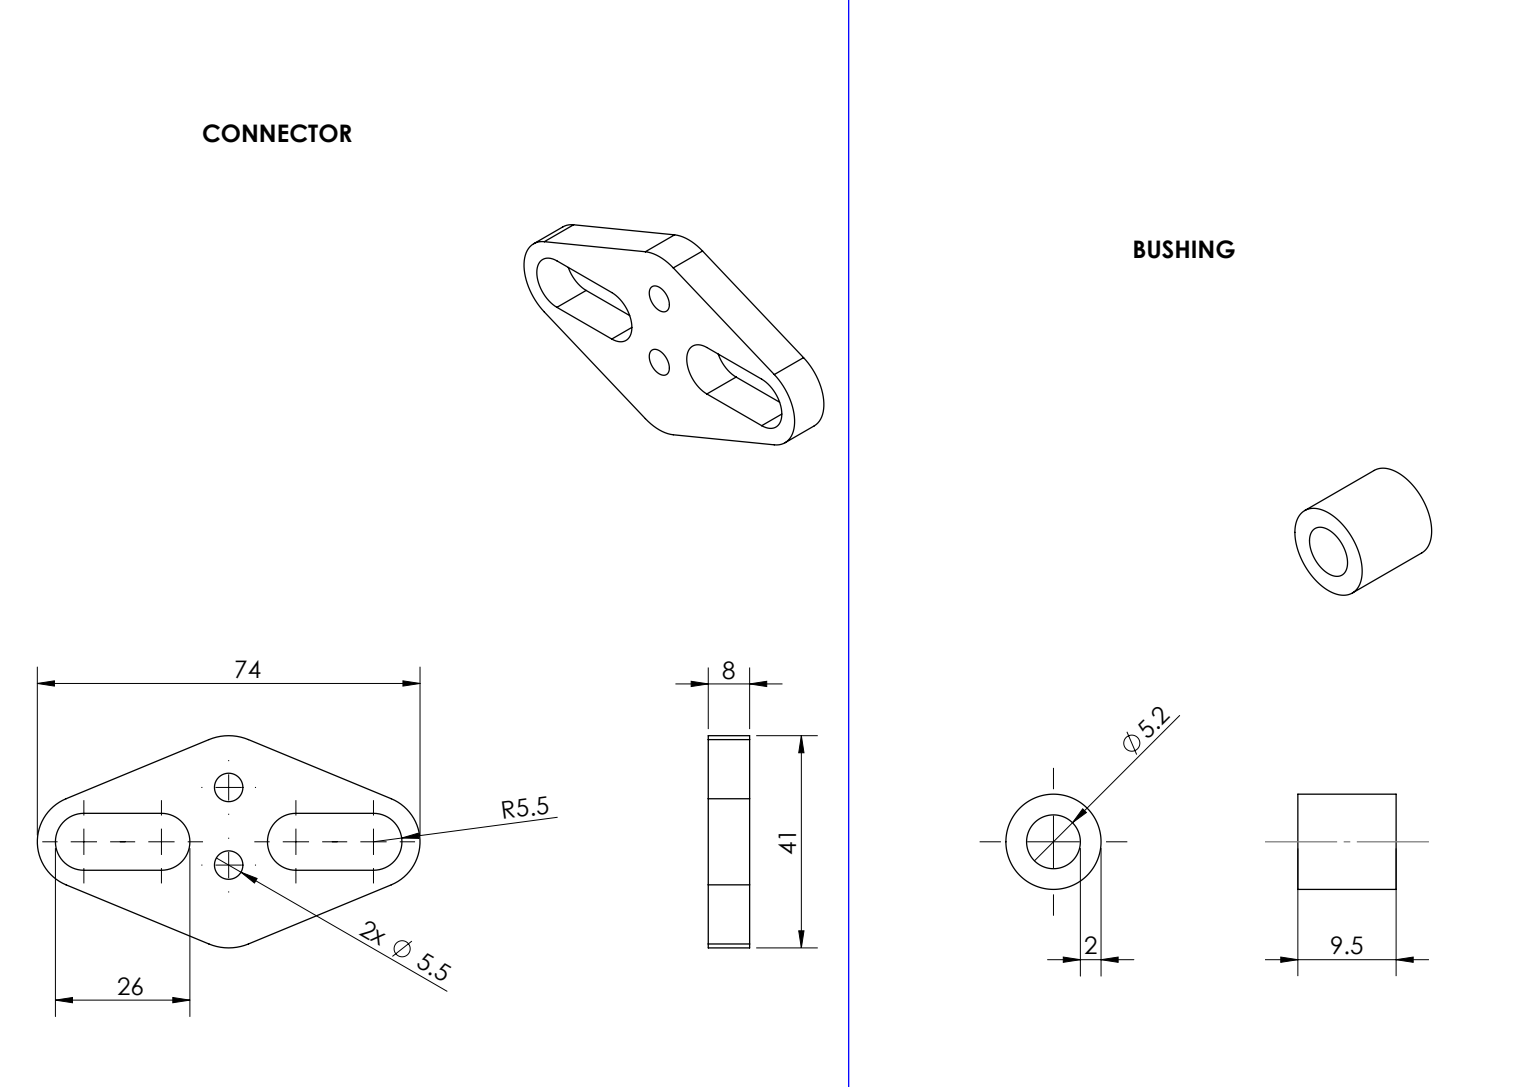
ISO-10303-21;
HEADER;
FILE_DESCRIPTION (('STEP AP214'),
    '1' );
FILE_NAME ('bushing.step',
    '2026-09-24T10:26:00',
    ( '' ),
    ( '' ),
    'SwSTEP 2.0',
    'SolidWorks 2026',
    '' );
FILE_SCHEMA (( 'AUTOMOTIVE_DESIGN' ));
ENDSEC;

DATA;
#17=EDGE_CURVE ( 'NONE', #13288, #10667, #2123, .T. ) ;
#63=PRODUCT ( 'bushing', 'bushing', '', ( #1978 ) ) ;
#90=SURFACE_STYLE_FILL_AREA ( #4690 ) ;
#131=VERTEX_POINT ( 'NONE', #10090 ) ;
#167=CARTESIAN_POINT ( 'NONE',  ( 0.000000000000000000, 0.000000000000000000, 0.000000000000000000 ) ) ;
#198=LINE ( 'NONE', #5806, #5338 ) ;
#221=AXIS2_PLACEMENT_3D ( 'NONE', #6634, #1226, #3433 ) ;
#307=UNCERTAINTY_MEASURE_WITH_UNIT (LENGTH_MEASURE( 1.000000000000000082E-05 ), #6803, 'distance_accuracy_value', 'NONE');
#327=EDGE_CURVE ( 'NONE', #12296, #10667, #14351, .T. ) ;
#475=SURFACE_STYLE_FILL_AREA ( #10569 ) ;
#957=AXIS2_PLACEMENT_3D ( 'NONE', #1843, #13854, #8266 ) ;
#1044=PRODUCT_DEFINITION_CONTEXT ( 'detailed design', #12786, 'design' ) ;
#1088=EDGE_CURVE ( 'NONE', #10667, #12296, #12886, .T. ) ;
#1201=( GEOMETRIC_REPRESENTATION_CONTEXT ( 3 ) GLOBAL_UNCERTAINTY_ASSIGNED_CONTEXT ( ( #8054 ) ) GLOBAL_UNIT_ASSIGNED_CONTEXT ( ( #10718, #4082, #12760 ) ) REPRESENTATION_CONTEXT ( 'NONE', 'WORKASPACE' ) );
#1226=DIRECTION ( 'NONE',  ( 0.000000000000000000, 0.000000000000000000, -1.000000000000000000 ) ) ;
#1235=EDGE_CURVE ( 'NONE', #14042, #13288, #9119, .T. ) ;
#1400=SHAPE_REPRESENTATION ( 'bushing', ( #11025 ), #4496 ) ;
#1424=AXIS2_PLACEMENT_3D ( 'NONE', #12440, #8035, #12508 ) ;
#1490=PLANE ( 'NONE',  #4984 ) ;
#1555=EDGE_CURVE ( 'NONE', #8738, #12036, #8933, .T. ) ;
#1727=EDGE_CURVE ( 'NONE', #8738, #13954, #7266, .T. ) ;
#1833=CYLINDRICAL_SURFACE ( 'NONE', #4021, 4.599999999999999645 ) ;
#1843=CARTESIAN_POINT ( 'NONE',  ( 28.00000000000000355, 29.99999999999999645, -34.50000000000000000 ) ) ;
#1978=PRODUCT_CONTEXT ( 'NONE', #7358, 'mechanical' ) ;
#1980=DIRECTION ( 'NONE',  ( 0.000000000000000000, 0.000000000000000000, -1.000000000000000000 ) ) ;
#2067=DIRECTION ( 'NONE',  ( -1.000000000000000000, 0.000000000000000000, 0.000000000000000000 ) ) ;
#2122=ORIENTED_EDGE ( 'NONE', *, *, #327, .F. ) ;
#2123=LINE ( 'NONE', #12076, #5253 ) ;
#2130=CARTESIAN_POINT ( 'NONE',  ( 30.60000000000000853, 29.99999999999999645, -24.99999999999999289 ) ) ;
#2532=ORIENTED_EDGE ( 'NONE', *, *, #4053, .F. ) ;
#2637=FACE_OUTER_BOUND ( 'NONE', #10692, .T. ) ;
#2660=CARTESIAN_POINT ( 'NONE',  ( 32.60000000000000142, 29.99999999999999645, -34.50000000000000000 ) ) ;
#2840=DIRECTION ( 'NONE',  ( 0.000000000000000000, 0.000000000000000000, -1.000000000000000000 ) ) ;
#2852=STYLED_ITEM ( 'NONE', ( #9618 ), #11938 ) ;
#2947=CARTESIAN_POINT ( 'NONE',  ( 28.00000000000000355, 29.99999999999999645, -34.50000000000000000 ) ) ;
#3172=EDGE_CURVE ( 'NONE', #14042, #12296, #5144, .T. ) ;
#3238=CARTESIAN_POINT ( 'NONE',  ( 23.40000000000000213, 29.99999999999999645, -24.99999999999999289 ) ) ;
#3381=( GEOMETRIC_REPRESENTATION_CONTEXT ( 3 ) GLOBAL_UNCERTAINTY_ASSIGNED_CONTEXT ( ( #307 ) ) GLOBAL_UNIT_ASSIGNED_CONTEXT ( ( #6803, #13337, #12303 ) ) REPRESENTATION_CONTEXT ( 'NONE', 'WORKASPACE' ) );
#3390=SURFACE_SIDE_STYLE ('',( #90 ) ) ;
#3399=DIRECTION ( 'NONE',  ( 0.000000000000000000, 0.000000000000000000, 1.000000000000000000 ) ) ;
#3433=DIRECTION ( 'NONE',  ( -1.000000000000000000, 0.000000000000000000, 0.000000000000000000 ) ) ;
#3454=FILL_AREA_STYLE_COLOUR ( '', #12640 ) ;
#3476=ADVANCED_FACE ( 'NONE', ( #3864, #3644 ), #3788, .F. ) ;
#3545=ORIENTED_EDGE ( 'NONE', *, *, #1555, .T. ) ;
#3554=UNCERTAINTY_MEASURE_WITH_UNIT (LENGTH_MEASURE( 1.000000000000000082E-05 ), #6295, 'distance_accuracy_value', 'NONE');
#3644=FACE_BOUND ( 'NONE', #8759, .T. ) ;
#3688=CARTESIAN_POINT ( 'NONE',  ( 28.00000000000000355, 29.99999999999999645, -24.99999999999999289 ) ) ;
#3750=ADVANCED_FACE ( 'NONE', ( #7708, #3845 ), #1490, .T. ) ;
#3788=PLANE ( 'NONE',  #5864 ) ;
#3845=FACE_BOUND ( 'NONE', #6428, .T. ) ;
#3864=FACE_OUTER_BOUND ( 'NONE', #10022, .T. ) ;
#3952=ORIENTED_EDGE ( 'NONE', *, *, #17, .T. ) ;
#3999=EDGE_LOOP ( 'NONE', ( #5182, #7262, #9638, #5982 ) ) ;
#4021=AXIS2_PLACEMENT_3D ( 'NONE', #2947, #8699, #12005 ) ;
#4053=EDGE_CURVE ( 'NONE', #12036, #131, #12295, .T. ) ;
#4076=DIRECTION ( 'NONE',  ( 1.000000000000000000, 0.000000000000000000, 0.000000000000000000 ) ) ;
#4082=( NAMED_UNIT ( * ) PLANE_ANGLE_UNIT ( ) SI_UNIT ( $, .RADIAN. ) );
#4139=CARTESIAN_POINT ( 'NONE',  ( 28.00000000000000355, 29.99999999999999645, -34.50000000000000000 ) ) ;
#4242=DIRECTION ( 'NONE',  ( 0.000000000000000000, 0.000000000000000000, -1.000000000000000000 ) ) ;
#4416=ORIENTED_EDGE ( 'NONE', *, *, #4053, .T. ) ;
#4496=( GEOMETRIC_REPRESENTATION_CONTEXT ( 3 ) GLOBAL_UNCERTAINTY_ASSIGNED_CONTEXT ( ( #3554 ) ) GLOBAL_UNIT_ASSIGNED_CONTEXT ( ( #6295, #13197, #5205 ) ) REPRESENTATION_CONTEXT ( 'NONE', 'WORKASPACE' ) );
#4503=DIRECTION ( 'NONE',  ( -1.000000000000000000, 0.000000000000000000, 0.000000000000000000 ) ) ;
#4611=VECTOR ( 'NONE', #10707, 1000.000000000000000 ) ;
#4642=AXIS2_PLACEMENT_3D ( 'NONE', #7297, #4242, #11772 ) ;
#4670=DIRECTION ( 'NONE',  ( 0.000000000000000000, 0.000000000000000000, 1.000000000000000000 ) ) ;
#4690=FILL_AREA_STYLE ('',( #3454 ) ) ;
#4870=ORIENTED_EDGE ( 'NONE', *, *, #1088, .F. ) ;
#4945=ORIENTED_EDGE ( 'NONE', *, *, #3172, .F. ) ;
#4984=AXIS2_PLACEMENT_3D ( 'NONE', #5856, #5933, #12751 ) ;
#5009=CARTESIAN_POINT ( 'NONE',  ( 28.00000000000000355, 29.99999999999999645, -34.50000000000000000 ) ) ;
#5142=DIRECTION ( 'NONE',  ( 0.000000000000000000, 0.000000000000000000, -1.000000000000000000 ) ) ;
#5144=LINE ( 'NONE', #11885, #4611 ) ;
#5155=AXIS2_PLACEMENT_3D ( 'NONE', #5009, #14095, #4076 ) ;
#5181=DIRECTION ( 'NONE',  ( -1.000000000000000000, 0.000000000000000000, 0.000000000000000000 ) ) ;
#5182=ORIENTED_EDGE ( 'NONE', *, *, #1555, .F. ) ;
#5205=( NAMED_UNIT ( * ) SI_UNIT ( $, .STERADIAN. ) SOLID_ANGLE_UNIT ( ) );
#5252=DIRECTION ( 'NONE',  ( 0.000000000000000000, 0.000000000000000000, 1.000000000000000000 ) ) ;
#5253=VECTOR ( 'NONE', #13119, 1000.000000000000000 ) ;
#5338=VECTOR ( 'NONE', #4670, 1000.000000000000000 ) ;
#5441=DIRECTION ( 'NONE',  ( 1.000000000000000000, 0.000000000000000000, 0.000000000000000000 ) ) ;
#5457=AXIS2_PLACEMENT_3D ( 'NONE', #6271, #7371, #5181 ) ;
#5565=ADVANCED_BREP_SHAPE_REPRESENTATION ( '', ( #11938, #11025 ), #4496 ) ;
#5623=AXIS2_PLACEMENT_3D ( 'NONE', #4139, #5142, #2067 ) ;
#5752=CYLINDRICAL_SURFACE ( 'NONE', #1424, 2.600000000000004974 ) ;
#5806=CARTESIAN_POINT ( 'NONE',  ( 32.60000000000000142, 29.99999999999999645, -34.50000000000000000 ) ) ;
#5856=CARTESIAN_POINT ( 'NONE',  ( 28.00000000000000355, 29.99999999999999645, -34.50000000000000000 ) ) ;
#5864=AXIS2_PLACEMENT_3D ( 'NONE', #8298, #2840, #12549 ) ;
#5915=MECHANICAL_DESIGN_GEOMETRIC_PRESENTATION_REPRESENTATION('',(#12250),#3381);
#5933=DIRECTION ( 'NONE',  ( 0.000000000000000000, 0.000000000000000000, -1.000000000000000000 ) ) ;
#5982=ORIENTED_EDGE ( 'NONE', *, *, #6678, .T. ) ;
#6199=ADVANCED_FACE ( 'NONE', ( #8434 ), #8281, .F. ) ;
#6271=CARTESIAN_POINT ( 'NONE',  ( 28.00000000000000355, 29.99999999999999645, -24.99999999999999289 ) ) ;
#6295=( LENGTH_UNIT ( ) NAMED_UNIT ( * ) SI_UNIT ( .MILLI., .METRE. ) );
#6337=ORIENTED_EDGE ( 'NONE', *, *, #6678, .F. ) ;
#6353=SHAPE_DEFINITION_REPRESENTATION ( #13869, #1400 ) ;
#6355=CARTESIAN_POINT ( 'NONE',  ( 28.00000000000000355, 29.99999999999999645, -34.50000000000000000 ) ) ;
#6428=EDGE_LOOP ( 'NONE', ( #11229, #10714 ) ) ;
#6470=CARTESIAN_POINT ( 'NONE',  ( 28.00000000000000355, 29.99999999999999645, -34.50000000000000000 ) ) ;
#6497=CIRCLE ( 'NONE', #4642, 2.600000000000004974 ) ;
#6524=DIRECTION ( 'NONE',  ( 0.000000000000000000, 0.000000000000000000, 1.000000000000000000 ) ) ;
#6634=CARTESIAN_POINT ( 'NONE',  ( 28.00000000000000355, 29.99999999999999645, -24.99999999999999289 ) ) ;
#6678=EDGE_CURVE ( 'NONE', #131, #12036, #11918, .T. ) ;
#6740=DIRECTION ( 'NONE',  ( 0.000000000000000000, 0.000000000000000000, -1.000000000000000000 ) ) ;
#6803=( LENGTH_UNIT ( ) NAMED_UNIT ( * ) SI_UNIT ( .MILLI., .METRE. ) );
#6976=ORIENTED_EDGE ( 'NONE', *, *, #8145, .T. ) ;
#7154=CARTESIAN_POINT ( 'NONE',  ( 30.60000000000000853, 29.99999999999999645, -34.50000000000000000 ) ) ;
#7196=AXIS2_PLACEMENT_3D ( 'NONE', #6470, #5252, #14258 ) ;
#7262=ORIENTED_EDGE ( 'NONE', *, *, #12274, .F. ) ;
#7266=CIRCLE ( 'NONE', #957, 4.600000000000003197 ) ;
#7297=CARTESIAN_POINT ( 'NONE',  ( 28.00000000000000355, 29.99999999999999645, -34.50000000000000000 ) ) ;
#7358=APPLICATION_CONTEXT ( 'automotive_design' ) ;
#7371=DIRECTION ( 'NONE',  ( 0.000000000000000000, 0.000000000000000000, -1.000000000000000000 ) ) ;
#7574=FACE_OUTER_BOUND ( 'NONE', #7896, .T. ) ;
#7708=FACE_OUTER_BOUND ( 'NONE', #12814, .T. ) ;
#7814=CLOSED_SHELL ( 'NONE', ( #6199, #8249, #3750, #3476, #12271, #10814 ) ) ;
#7896=EDGE_LOOP ( 'NONE', ( #13674, #3545, #4416, #9519 ) ) ;
#8013=PRODUCT_DEFINITION ( 'UNKNOWN', '', #14355, #1044 ) ;
#8035=DIRECTION ( 'NONE',  ( 0.000000000000000000, 0.000000000000000000, 1.000000000000000000 ) ) ;
#8038=SHAPE_REPRESENTATION_RELATIONSHIP ( 'NONE' , 'NONE' ,  #1400, #5565 ) ;
#8054=UNCERTAINTY_MEASURE_WITH_UNIT (LENGTH_MEASURE( 1.000000000000000082E-05 ), #10718, 'distance_accuracy_value', 'NONE');
#8094=ORIENTED_EDGE ( 'NONE', *, *, #1727, .T. ) ;
#8145=EDGE_CURVE ( 'NONE', #13288, #14042, #6497, .T. ) ;
#8249=ADVANCED_FACE ( 'NONE', ( #7574 ), #14052, .T. ) ;
#8266=DIRECTION ( 'NONE',  ( -1.000000000000000000, 0.000000000000000000, 0.000000000000000000 ) ) ;
#8281=CYLINDRICAL_SURFACE ( 'NONE', #5155, 2.600000000000004974 ) ;
#8298=CARTESIAN_POINT ( 'NONE',  ( 28.00000000000000355, 29.99999999999999645, -24.99999999999999289 ) ) ;
#8434=FACE_OUTER_BOUND ( 'NONE', #13665, .T. ) ;
#8529=ORIENTED_EDGE ( 'NONE', *, *, #1088, .T. ) ;
#8659=ORIENTED_EDGE ( 'NONE', *, *, #3172, .T. ) ;
#8699=DIRECTION ( 'NONE',  ( 0.000000000000000000, 0.000000000000000000, 1.000000000000000000 ) ) ;
#8738=VERTEX_POINT ( 'NONE', #13688 ) ;
#8759=EDGE_LOOP ( 'NONE', ( #8529, #10054 ) ) ;
#8782=SURFACE_SIDE_STYLE ('',( #475 ) ) ;
#8933=LINE ( 'NONE', #13430, #13600 ) ;
#9119=CIRCLE ( 'NONE', #5623, 2.600000000000004974 ) ;
#9127=COLOUR_RGB ( '', 0.31764706, 0.68627451, 0.89019608) ;
#9139=MECHANICAL_DESIGN_GEOMETRIC_PRESENTATION_REPRESENTATION('',(#2852),#1201);
#9275=EDGE_CURVE ( 'NONE', #13954, #131, #198, .T. ) ;
#9394=SURFACE_STYLE_USAGE ( .BOTH. , #8782 ) ;
#9519=ORIENTED_EDGE ( 'NONE', *, *, #9275, .F. ) ;
#9618=PRESENTATION_STYLE_ASSIGNMENT (( #9394 ) ) ;
#9638=ORIENTED_EDGE ( 'NONE', *, *, #9275, .T. ) ;
#10022=EDGE_LOOP ( 'NONE', ( #6337, #2532 ) ) ;
#10054=ORIENTED_EDGE ( 'NONE', *, *, #327, .T. ) ;
#10090=CARTESIAN_POINT ( 'NONE',  ( 32.60000000000000142, 29.99999999999999645, -24.99999999999999289 ) ) ;
#10170=SURFACE_STYLE_USAGE ( .BOTH. , #3390 ) ;
#10493=FILL_AREA_STYLE_COLOUR ( '', #9127 ) ;
#10559=DIRECTION ( 'NONE',  ( 0.000000000000000000, 0.000000000000000000, -1.000000000000000000 ) ) ;
#10569=FILL_AREA_STYLE ('',( #10493 ) ) ;
#10667=VERTEX_POINT ( 'NONE', #2130 ) ;
#10692=EDGE_LOOP ( 'NONE', ( #4945, #11673, #3952, #2122 ) ) ;
#10707=DIRECTION ( 'NONE',  ( 0.000000000000000000, 0.000000000000000000, 1.000000000000000000 ) ) ;
#10714=ORIENTED_EDGE ( 'NONE', *, *, #1235, .F. ) ;
#10718=( LENGTH_UNIT ( ) NAMED_UNIT ( * ) SI_UNIT ( .MILLI., .METRE. ) );
#10814=ADVANCED_FACE ( 'NONE', ( #2637 ), #5752, .F. ) ;
#10821=ORIENTED_EDGE ( 'NONE', *, *, #12274, .T. ) ;
#11025=AXIS2_PLACEMENT_3D ( 'NONE', #167, #6524, #5441 ) ;
#11135=CARTESIAN_POINT ( 'NONE',  ( 28.00000000000000355, 29.99999999999999645, -24.99999999999999289 ) ) ;
#11229=ORIENTED_EDGE ( 'NONE', *, *, #8145, .F. ) ;
#11673=ORIENTED_EDGE ( 'NONE', *, *, #1235, .T. ) ;
#11723=AXIS2_PLACEMENT_3D ( 'NONE', #6355, #1980, #14205 ) ;
#11772=DIRECTION ( 'NONE',  ( -1.000000000000000000, 0.000000000000000000, 0.000000000000000000 ) ) ;
#11885=CARTESIAN_POINT ( 'NONE',  ( 25.39999999999999858, 29.99999999999999645, -34.50000000000000000 ) ) ;
#11918=CIRCLE ( 'NONE', #221, 4.600000000000003197 ) ;
#11938=MANIFOLD_SOLID_BREP ( 'Extrude-Thin1', #7814 ) ;
#11956=ORIENTED_EDGE ( 'NONE', *, *, #17, .F. ) ;
#12005=DIRECTION ( 'NONE',  ( 1.000000000000000000, 0.000000000000000000, 0.000000000000000000 ) ) ;
#12036=VERTEX_POINT ( 'NONE', #3238 ) ;
#12076=CARTESIAN_POINT ( 'NONE',  ( 30.60000000000000853, 29.99999999999999645, -34.50000000000000000 ) ) ;
#12182=CIRCLE ( 'NONE', #11723, 4.600000000000003197 ) ;
#12250=STYLED_ITEM ( 'NONE', ( #13631 ), #5565 ) ;
#12271=ADVANCED_FACE ( 'NONE', ( #14068 ), #1833, .T. ) ;
#12274=EDGE_CURVE ( 'NONE', #13954, #8738, #12182, .T. ) ;
#12295=CIRCLE ( 'NONE', #14402, 4.600000000000003197 ) ;
#12296=VERTEX_POINT ( 'NONE', #12887 ) ;
#12303=( NAMED_UNIT ( * ) SI_UNIT ( $, .STERADIAN. ) SOLID_ANGLE_UNIT ( ) );
#12440=CARTESIAN_POINT ( 'NONE',  ( 28.00000000000000355, 29.99999999999999645, -34.50000000000000000 ) ) ;
#12508=DIRECTION ( 'NONE',  ( 1.000000000000000000, 0.000000000000000000, 0.000000000000000000 ) ) ;
#12549=DIRECTION ( 'NONE',  ( -1.000000000000000000, 0.000000000000000000, 0.000000000000000000 ) ) ;
#12632=AXIS2_PLACEMENT_3D ( 'NONE', #3688, #10559, #12831 ) ;
#12640=COLOUR_RGB ( '', 0.31764706, 0.68627451, 0.89019608) ;
#12751=DIRECTION ( 'NONE',  ( -1.000000000000000000, 0.000000000000000000, 0.000000000000000000 ) ) ;
#12760=( NAMED_UNIT ( * ) SI_UNIT ( $, .STERADIAN. ) SOLID_ANGLE_UNIT ( ) );
#12786=APPLICATION_CONTEXT ( 'automotive_design' ) ;
#12814=EDGE_LOOP ( 'NONE', ( #10821, #8094 ) ) ;
#12831=DIRECTION ( 'NONE',  ( -1.000000000000000000, 0.000000000000000000, 0.000000000000000000 ) ) ;
#12886=CIRCLE ( 'NONE', #12632, 2.600000000000004974 ) ;
#12887=CARTESIAN_POINT ( 'NONE',  ( 25.39999999999999858, 29.99999999999999645, -24.99999999999999289 ) ) ;
#13119=DIRECTION ( 'NONE',  ( 0.000000000000000000, 0.000000000000000000, 1.000000000000000000 ) ) ;
#13197=( NAMED_UNIT ( * ) PLANE_ANGLE_UNIT ( ) SI_UNIT ( $, .RADIAN. ) );
#13288=VERTEX_POINT ( 'NONE', #7154 ) ;
#13337=( NAMED_UNIT ( * ) PLANE_ANGLE_UNIT ( ) SI_UNIT ( $, .RADIAN. ) );
#13430=CARTESIAN_POINT ( 'NONE',  ( 23.40000000000000213, 29.99999999999999645, -34.50000000000000000 ) ) ;
#13600=VECTOR ( 'NONE', #3399, 1000.000000000000000 ) ;
#13631=PRESENTATION_STYLE_ASSIGNMENT (( #10170 ) ) ;
#13665=EDGE_LOOP ( 'NONE', ( #6976, #8659, #4870, #11956 ) ) ;
#13674=ORIENTED_EDGE ( 'NONE', *, *, #1727, .F. ) ;
#13688=CARTESIAN_POINT ( 'NONE',  ( 23.40000000000000213, 29.99999999999999645, -34.50000000000000000 ) ) ;
#13854=DIRECTION ( 'NONE',  ( 0.000000000000000000, 0.000000000000000000, -1.000000000000000000 ) ) ;
#13869=PRODUCT_DEFINITION_SHAPE ( 'NONE', 'NONE',  #8013 ) ;
#13954=VERTEX_POINT ( 'NONE', #2660 ) ;
#14042=VERTEX_POINT ( 'NONE', #14153 ) ;
#14052=CYLINDRICAL_SURFACE ( 'NONE', #7196, 4.599999999999999645 ) ;
#14068=FACE_OUTER_BOUND ( 'NONE', #3999, .T. ) ;
#14095=DIRECTION ( 'NONE',  ( 0.000000000000000000, 0.000000000000000000, 1.000000000000000000 ) ) ;
#14153=CARTESIAN_POINT ( 'NONE',  ( 25.39999999999999858, 29.99999999999999645, -34.50000000000000000 ) ) ;
#14205=DIRECTION ( 'NONE',  ( -1.000000000000000000, 0.000000000000000000, 0.000000000000000000 ) ) ;
#14258=DIRECTION ( 'NONE',  ( 1.000000000000000000, 0.000000000000000000, 0.000000000000000000 ) ) ;
#14351=CIRCLE ( 'NONE', #5457, 2.600000000000004974 ) ;
#14355=PRODUCT_DEFINITION_FORMATION_WITH_SPECIFIED_SOURCE ( 'ANY', '', #63, .NOT_KNOWN. ) ;
#14402=AXIS2_PLACEMENT_3D ( 'NONE', #11135, #6740, #4503 ) ;
ENDSEC;
END-ISO-10303-21;
